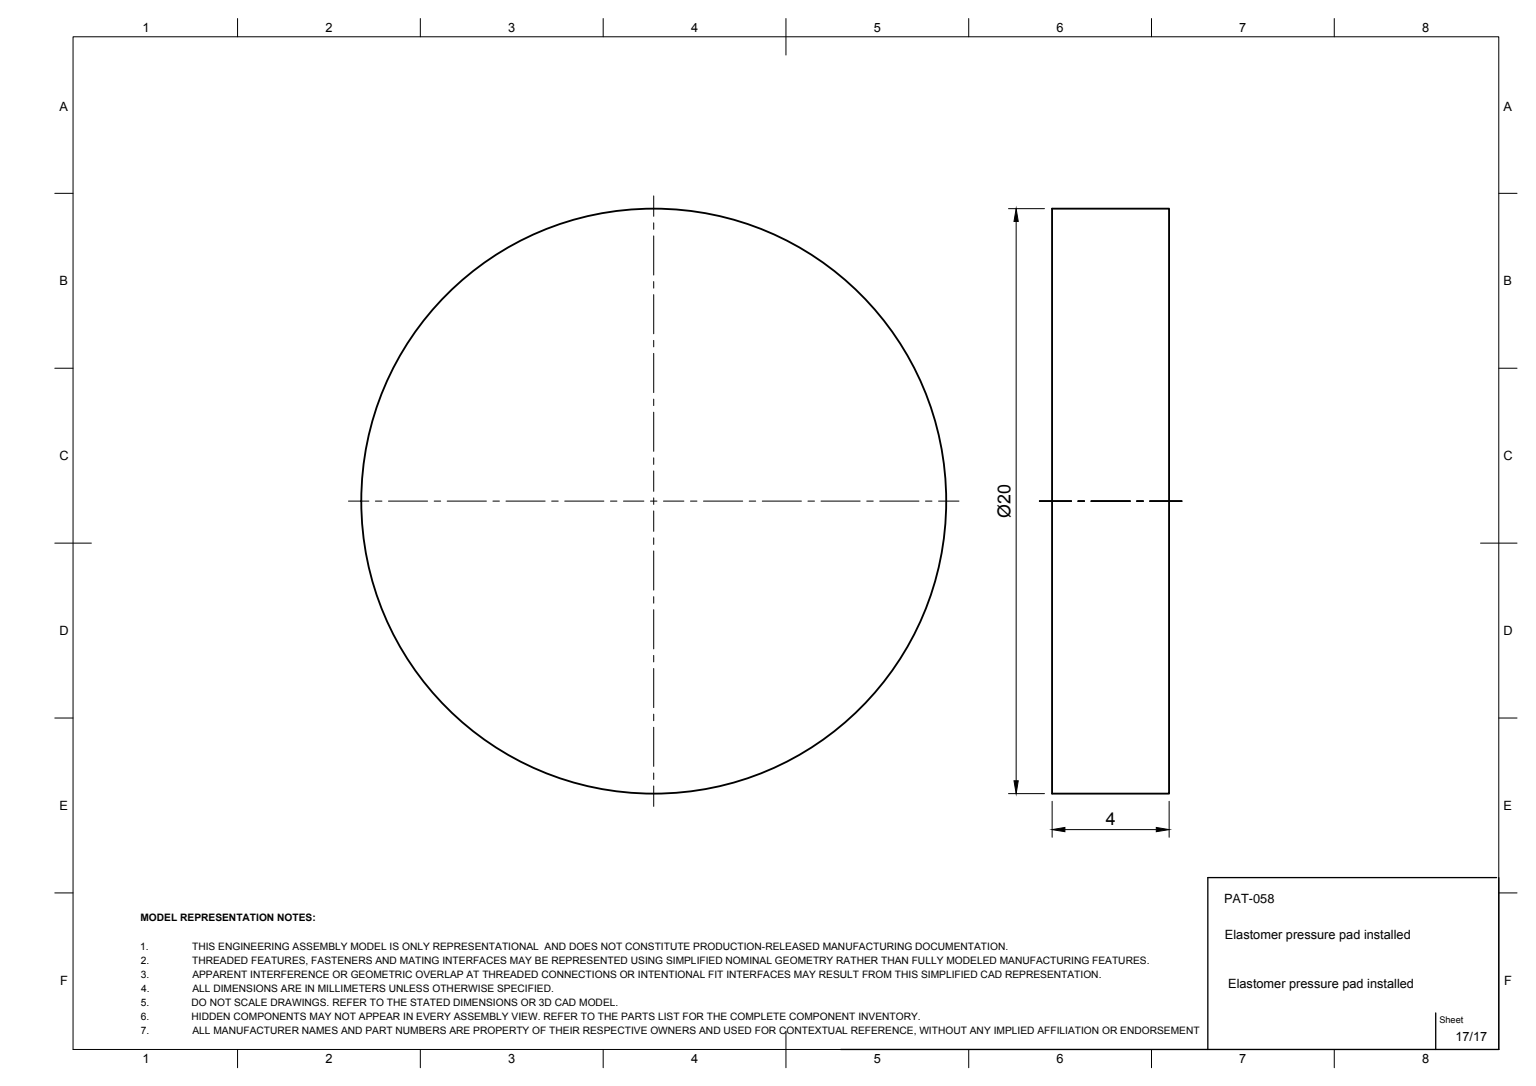
ISO-10303-21;
HEADER;
/* Generated by software containing ST-Developer
 * from STEP Tools, Inc. (www.steptools.com) 
 */

FILE_DESCRIPTION(
/* description */ ('Horizontal push-pull toggle clamp'),
/* implementation_level */ '2;1');

FILE_NAME(
/* name */ 'Elastomer pressure pad installed.step',
/* time_stamp */ '2026-10-27T21:21:09-07:00',
/* author */ (''),
/* organization */ (''),
/* preprocessor_version */ 'ST-DEVELOPER v20.2',
/* originating_system */ 'Autodesk Translation Framework v15.17.0.0',
/* authorisation */ '');

FILE_SCHEMA (('AUTOMOTIVE_DESIGN { 1 0 10303 214 3 1 1 }'));
ENDSEC;

DATA;
#10=MECHANICAL_DESIGN_GEOMETRIC_PRESENTATION_REPRESENTATION('',(#193),#4791);
#167=SHAPE_REPRESENTATION_RELATIONSHIP('SRR','None',#4873,#180);
#180=ADVANCED_BREP_SHAPE_REPRESENTATION('',(#205),#4786);
#193=STYLED_ITEM('',(#5037),#205);
#205=MANIFOLD_SOLID_BREP('Body1',#2638);
#350=PLANE('',#2997);
#351=PLANE('',#2998);
#489=FACE_OUTER_BOUND('',#679,.T.);
#490=FACE_OUTER_BOUND('',#680,.T.);
#491=FACE_OUTER_BOUND('',#681,.T.);
#679=EDGE_LOOP('',(#2357,#2358,#2359,#2360));
#680=EDGE_LOOP('',(#2361));
#681=EDGE_LOOP('',(#2362));
#775=CIRCLE('',#2995,1.);
#776=CIRCLE('',#2996,1.);
#1000=LINE('',#4514,#1220);
#1220=VECTOR('',#3692,1.);
#1425=VERTEX_POINT('',#4511);
#1426=VERTEX_POINT('',#4513);
#1740=EDGE_CURVE('',#1425,#1425,#775,.T.);
#1741=EDGE_CURVE('',#1425,#1426,#1000,.T.);
#1742=EDGE_CURVE('',#1426,#1426,#776,.T.);
#2357=ORIENTED_EDGE('',*,*,#1740,.F.);
#2358=ORIENTED_EDGE('',*,*,#1741,.T.);
#2359=ORIENTED_EDGE('',*,*,#1742,.T.);
#2360=ORIENTED_EDGE('',*,*,#1741,.F.);
#2361=ORIENTED_EDGE('',*,*,#1740,.T.);
#2362=ORIENTED_EDGE('',*,*,#1742,.F.);
#2469=CYLINDRICAL_SURFACE('',#2994,1.);
#2605=ADVANCED_FACE('',(#489),#2469,.T.);
#2606=ADVANCED_FACE('',(#490),#350,.T.);
#2607=ADVANCED_FACE('',(#491),#351,.F.);
#2638=CLOSED_SHELL('',(#2605,#2606,#2607));
#2993=AXIS2_PLACEMENT_3D('',#4509,#3686,#3687);
#2994=AXIS2_PLACEMENT_3D('',#4510,#3688,#3689);
#2995=AXIS2_PLACEMENT_3D('',#4512,#3690,#3691);
#2996=AXIS2_PLACEMENT_3D('',#4515,#3693,#3694);
#2997=AXIS2_PLACEMENT_3D('',#4516,#3695,#3696);
#2998=AXIS2_PLACEMENT_3D('',#4517,#3697,#3698);
#3686=DIRECTION('axis',(0.,0.,1.));
#3687=DIRECTION('refdir',(1.,0.,0.));
#3688=DIRECTION('center_axis',(0.,0.,1.));
#3689=DIRECTION('ref_axis',(1.,0.,0.));
#3690=DIRECTION('center_axis',(0.,0.,1.));
#3691=DIRECTION('ref_axis',(1.,0.,0.));
#3692=DIRECTION('',(0.,0.,-1.));
#3693=DIRECTION('center_axis',(0.,0.,1.));
#3694=DIRECTION('ref_axis',(1.,0.,0.));
#3695=DIRECTION('center_axis',(0.,0.,1.));
#3696=DIRECTION('ref_axis',(1.,0.,0.));
#3697=DIRECTION('center_axis',(0.,0.,1.));
#3698=DIRECTION('ref_axis',(1.,0.,0.));
#4509=CARTESIAN_POINT('',(0.,0.,0.));
#4510=CARTESIAN_POINT('Origin',(0.,0.,3.));
#4511=CARTESIAN_POINT('',(-1.,-1.22464679914735E-16,3.4));
#4512=CARTESIAN_POINT('Origin',(0.,0.,3.4));
#4513=CARTESIAN_POINT('',(-1.,-1.22464679914735E-16,3.));
#4514=CARTESIAN_POINT('',(-1.,-1.22464679914735E-16,3.));
#4515=CARTESIAN_POINT('Origin',(0.,0.,3.));
#4516=CARTESIAN_POINT('Origin',(0.,0.,3.4));
#4517=CARTESIAN_POINT('Origin',(0.,0.,3.));
#4767=UNCERTAINTY_MEASURE_WITH_UNIT(LENGTH_MEASURE(0.001),#4792,
'DISTANCE_ACCURACY_VALUE',
'Maximum model space distance between geometric entities at asserted c
onnectivities');
#4772=UNCERTAINTY_MEASURE_WITH_UNIT(LENGTH_MEASURE(0.001),#4792,
'DISTANCE_ACCURACY_VALUE',
'Maximum model space distance between geometric entities at asserted c
onnectivities');
#4786=(
GEOMETRIC_REPRESENTATION_CONTEXT(3)
GLOBAL_UNCERTAINTY_ASSIGNED_CONTEXT((#4767))
GLOBAL_UNIT_ASSIGNED_CONTEXT((#4792,#4794,#4795))
REPRESENTATION_CONTEXT('','3D')
);
#4791=(
GEOMETRIC_REPRESENTATION_CONTEXT(3)
GLOBAL_UNCERTAINTY_ASSIGNED_CONTEXT((#4772))
GLOBAL_UNIT_ASSIGNED_CONTEXT((#4792,#4794,#4795))
REPRESENTATION_CONTEXT('','3D')
);
#4792=(
LENGTH_UNIT()
NAMED_UNIT(*)
SI_UNIT(.CENTI.,.METRE.)
);
#4794=(
NAMED_UNIT(*)
PLANE_ANGLE_UNIT()
SI_UNIT($,.RADIAN.)
);
#4795=(
NAMED_UNIT(*)
SI_UNIT($,.STERADIAN.)
SOLID_ANGLE_UNIT()
);
#4809=SHAPE_DEFINITION_REPRESENTATION(#4828,#4873);
#4828=PRODUCT_DEFINITION_SHAPE('',$,#4892);
#4873=SHAPE_REPRESENTATION('',(#2993),#4786);
#4878=PRODUCT_DEFINITION_CONTEXT('part definition',#4934,'design');
#4892=PRODUCT_DEFINITION('Elastomer pressure pad installed',
'Elastomer pressure pad installed',#4910,#4878);
#4910=PRODUCT_DEFINITION_FORMATION('',$,#4949);
#4934=APPLICATION_CONTEXT(
'Core Data for Automotive Mechanical Design Process');
#4935=PRODUCT_CONTEXT('part definition',#4934,'mechanical');
#4949=PRODUCT('Elastomer pressure pad installed',
'Elastomer pressure pad installed','Elastomer pressure pad installed',(#4935));
#5031=COLOUR_RGB('Off White',0.89,0.88,0.83);
#5032=FILL_AREA_STYLE_COLOUR('',#5031);
#5033=FILL_AREA_STYLE('',(#5032));
#5034=SURFACE_STYLE_FILL_AREA(#5033);
#5035=SURFACE_SIDE_STYLE('',(#5034));
#5036=SURFACE_STYLE_USAGE(.BOTH.,#5035);
#5037=PRESENTATION_STYLE_ASSIGNMENT((#5036));
ENDSEC;
END-ISO-10303-21;
